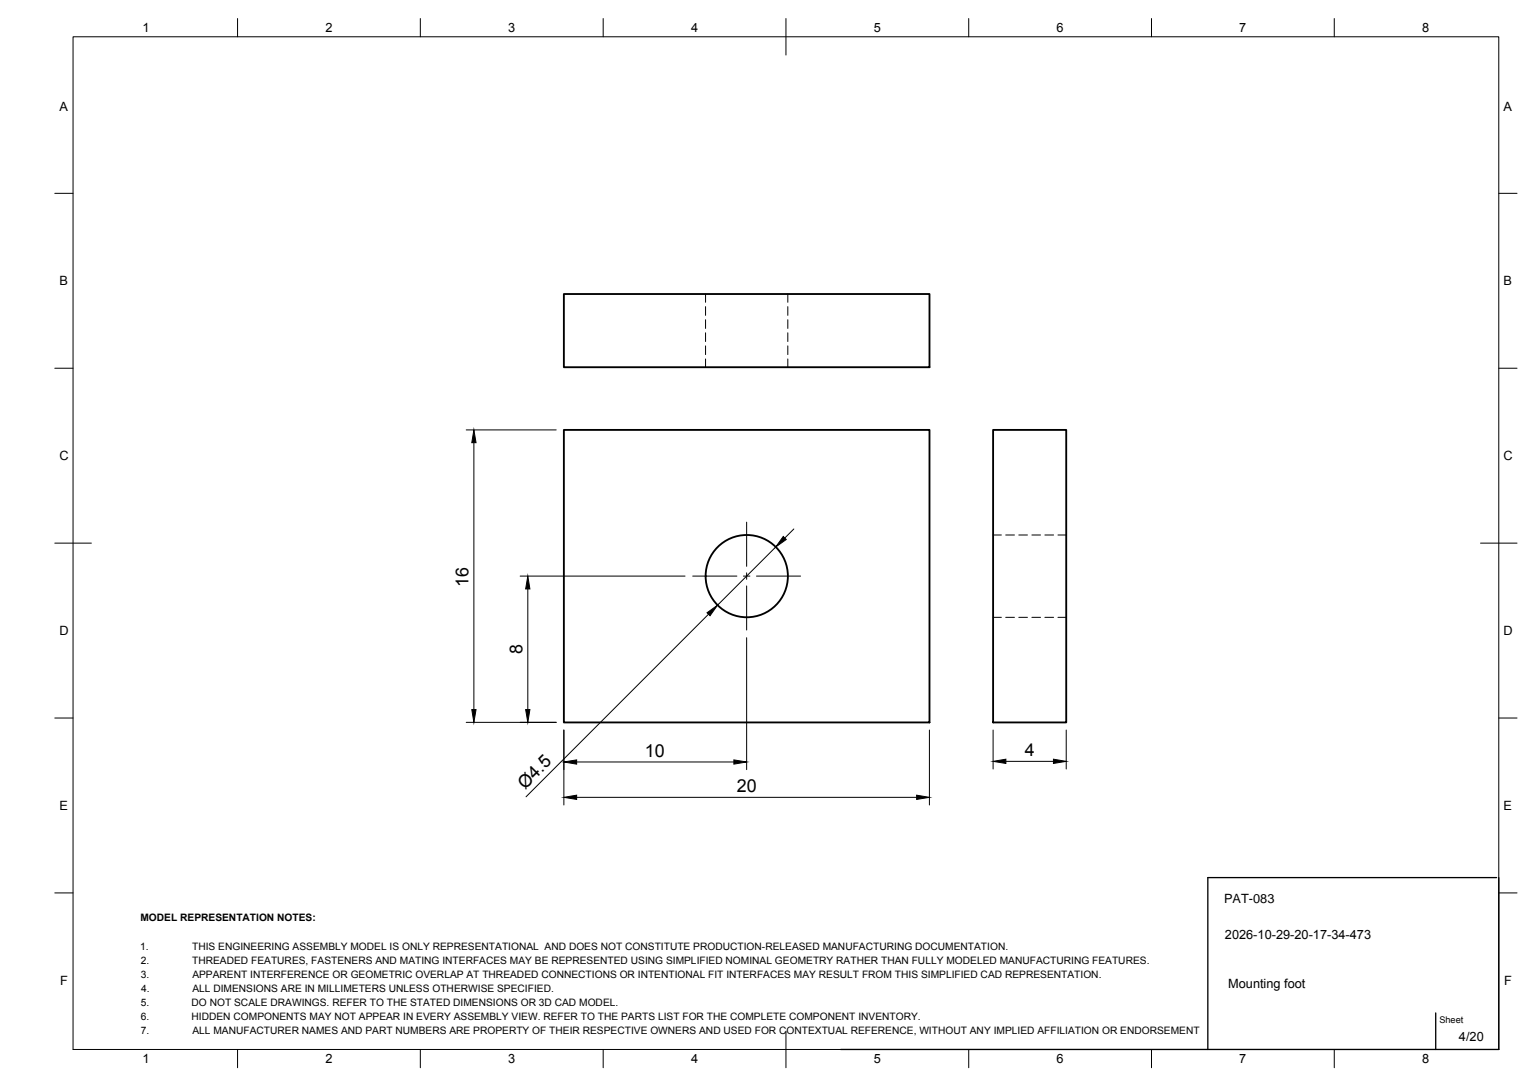
ISO-10303-21;
HEADER;
/* Generated by software containing ST-Developer
 * from STEP Tools, Inc. (www.steptools.com) 
 */

FILE_DESCRIPTION(
/* description */ ('PAT-083'),
/* implementation_level */ '2;1');

FILE_NAME(
/* name */ 'Mounting foot.step',
/* time_stamp */ '2026-10-29T20:18:00-07:00',
/* author */ (''),
/* organization */ (''),
/* preprocessor_version */ 'ST-DEVELOPER v20.2',
/* originating_system */ 'Autodesk Translation Framework v15.17.0.0',
/* authorisation */ '');

FILE_SCHEMA (('AUTOMOTIVE_DESIGN { 1 0 10303 214 3 1 1 }'));
ENDSEC;

DATA;
#10=MECHANICAL_DESIGN_GEOMETRIC_PRESENTATION_REPRESENTATION('',(#230),#8428);
#182=SHAPE_REPRESENTATION_RELATIONSHIP('SRR','None',#8516,#206);
#206=ADVANCED_BREP_SHAPE_REPRESENTATION('',(#254),#8405);
#230=STYLED_ITEM('',(#8698),#254);
#254=MANIFOLD_SOLID_BREP('Body1',#3676);
#279=FACE_BOUND('',#746,.T.);
#280=FACE_BOUND('',#748,.T.);
#362=PLANE('',#3984);
#363=PLANE('',#3985);
#364=PLANE('',#3986);
#365=PLANE('',#3987);
#366=PLANE('',#3988);
#367=PLANE('',#3989);
#503=FACE_OUTER_BOUND('',#740,.T.);
#504=FACE_OUTER_BOUND('',#741,.T.);
#505=FACE_OUTER_BOUND('',#742,.T.);
#506=FACE_OUTER_BOUND('',#743,.T.);
#507=FACE_OUTER_BOUND('',#744,.T.);
#508=FACE_OUTER_BOUND('',#745,.T.);
#509=FACE_OUTER_BOUND('',#747,.T.);
#740=EDGE_LOOP('',(#2494,#2495,#2496,#2497));
#741=EDGE_LOOP('',(#2498,#2499,#2500,#2501));
#742=EDGE_LOOP('',(#2502,#2503,#2504,#2505));
#743=EDGE_LOOP('',(#2506,#2507,#2508,#2509));
#744=EDGE_LOOP('',(#2510,#2511,#2512,#2513));
#745=EDGE_LOOP('',(#2514,#2515,#2516,#2517));
#746=EDGE_LOOP('',(#2518));
#747=EDGE_LOOP('',(#2519,#2520,#2521,#2522));
#748=EDGE_LOOP('',(#2523));
#1056=LINE('',#5665,#1300);
#1057=LINE('',#5670,#1301);
#1058=LINE('',#5672,#1302);
#1059=LINE('',#5674,#1303);
#1060=LINE('',#5675,#1304);
#1061=LINE('',#5678,#1305);
#1062=LINE('',#5680,#1306);
#1063=LINE('',#5681,#1307);
#1064=LINE('',#5684,#1308);
#1065=LINE('',#5686,#1309);
#1066=LINE('',#5687,#1310);
#1067=LINE('',#5689,#1311);
#1068=LINE('',#5690,#1312);
#1300=VECTOR('',#4484,0.225);
#1301=VECTOR('',#4489,1.);
#1302=VECTOR('',#4490,1.);
#1303=VECTOR('',#4491,1.);
#1304=VECTOR('',#4492,1.);
#1305=VECTOR('',#4495,1.);
#1306=VECTOR('',#4496,1.);
#1307=VECTOR('',#4497,1.);
#1308=VECTOR('',#4500,1.);
#1309=VECTOR('',#4501,1.);
#1310=VECTOR('',#4502,1.);
#1311=VECTOR('',#4505,1.);
#1312=VECTOR('',#4506,1.);
#1534=CIRCLE('',#3982,0.225);
#1535=CIRCLE('',#3983,0.225);
#1725=VERTEX_POINT('',#5662);
#1726=VERTEX_POINT('',#5664);
#1727=VERTEX_POINT('',#5668);
#1728=VERTEX_POINT('',#5669);
#1729=VERTEX_POINT('',#5671);
#1730=VERTEX_POINT('',#5673);
#1731=VERTEX_POINT('',#5677);
#1732=VERTEX_POINT('',#5679);
#1733=VERTEX_POINT('',#5683);
#1734=VERTEX_POINT('',#5685);
#2023=EDGE_CURVE('',#1725,#1725,#1534,.T.);
#2024=EDGE_CURVE('',#1725,#1726,#1056,.T.);
#2025=EDGE_CURVE('',#1726,#1726,#1535,.T.);
#2026=EDGE_CURVE('',#1727,#1728,#1057,.T.);
#2027=EDGE_CURVE('',#1728,#1729,#1058,.T.);
#2028=EDGE_CURVE('',#1730,#1729,#1059,.T.);
#2029=EDGE_CURVE('',#1727,#1730,#1060,.T.);
#2030=EDGE_CURVE('',#1731,#1727,#1061,.T.);
#2031=EDGE_CURVE('',#1732,#1730,#1062,.T.);
#2032=EDGE_CURVE('',#1731,#1732,#1063,.T.);
#2033=EDGE_CURVE('',#1733,#1731,#1064,.T.);
#2034=EDGE_CURVE('',#1734,#1732,#1065,.T.);
#2035=EDGE_CURVE('',#1733,#1734,#1066,.T.);
#2036=EDGE_CURVE('',#1728,#1733,#1067,.T.);
#2037=EDGE_CURVE('',#1729,#1734,#1068,.T.);
#2494=ORIENTED_EDGE('',*,*,#2023,.F.);
#2495=ORIENTED_EDGE('',*,*,#2024,.T.);
#2496=ORIENTED_EDGE('',*,*,#2025,.F.);
#2497=ORIENTED_EDGE('',*,*,#2024,.F.);
#2498=ORIENTED_EDGE('',*,*,#2026,.T.);
#2499=ORIENTED_EDGE('',*,*,#2027,.T.);
#2500=ORIENTED_EDGE('',*,*,#2028,.F.);
#2501=ORIENTED_EDGE('',*,*,#2029,.F.);
#2502=ORIENTED_EDGE('',*,*,#2030,.T.);
#2503=ORIENTED_EDGE('',*,*,#2029,.T.);
#2504=ORIENTED_EDGE('',*,*,#2031,.F.);
#2505=ORIENTED_EDGE('',*,*,#2032,.F.);
#2506=ORIENTED_EDGE('',*,*,#2033,.T.);
#2507=ORIENTED_EDGE('',*,*,#2032,.T.);
#2508=ORIENTED_EDGE('',*,*,#2034,.F.);
#2509=ORIENTED_EDGE('',*,*,#2035,.F.);
#2510=ORIENTED_EDGE('',*,*,#2036,.T.);
#2511=ORIENTED_EDGE('',*,*,#2035,.T.);
#2512=ORIENTED_EDGE('',*,*,#2037,.F.);
#2513=ORIENTED_EDGE('',*,*,#2027,.F.);
#2514=ORIENTED_EDGE('',*,*,#2037,.T.);
#2515=ORIENTED_EDGE('',*,*,#2034,.T.);
#2516=ORIENTED_EDGE('',*,*,#2031,.T.);
#2517=ORIENTED_EDGE('',*,*,#2028,.T.);
#2518=ORIENTED_EDGE('',*,*,#2025,.T.);
#2519=ORIENTED_EDGE('',*,*,#2036,.F.);
#2520=ORIENTED_EDGE('',*,*,#2026,.F.);
#2521=ORIENTED_EDGE('',*,*,#2030,.F.);
#2522=ORIENTED_EDGE('',*,*,#2033,.F.);
#2523=ORIENTED_EDGE('',*,*,#2023,.T.);
#3366=CYLINDRICAL_SURFACE('',#3981,0.225);
#3450=ADVANCED_FACE('',(#503),#3366,.F.);
#3451=ADVANCED_FACE('',(#504),#362,.T.);
#3452=ADVANCED_FACE('',(#505),#363,.T.);
#3453=ADVANCED_FACE('',(#506),#364,.T.);
#3454=ADVANCED_FACE('',(#507),#365,.T.);
#3455=ADVANCED_FACE('',(#508,#279),#366,.T.);
#3456=ADVANCED_FACE('',(#509,#280),#367,.F.);
#3676=CLOSED_SHELL('',(#3450,#3451,#3452,#3453,#3454,#3455,#3456));
#3980=AXIS2_PLACEMENT_3D('',#5660,#4478,#4479);
#3981=AXIS2_PLACEMENT_3D('',#5661,#4480,#4481);
#3982=AXIS2_PLACEMENT_3D('',#5663,#4482,#4483);
#3983=AXIS2_PLACEMENT_3D('',#5666,#4485,#4486);
#3984=AXIS2_PLACEMENT_3D('',#5667,#4487,#4488);
#3985=AXIS2_PLACEMENT_3D('',#5676,#4493,#4494);
#3986=AXIS2_PLACEMENT_3D('',#5682,#4498,#4499);
#3987=AXIS2_PLACEMENT_3D('',#5688,#4503,#4504);
#3988=AXIS2_PLACEMENT_3D('',#5691,#4507,#4508);
#3989=AXIS2_PLACEMENT_3D('',#5692,#4509,#4510);
#4478=DIRECTION('axis',(0.,0.,1.));
#4479=DIRECTION('refdir',(1.,0.,0.));
#4480=DIRECTION('center_axis',(0.,0.,1.));
#4481=DIRECTION('ref_axis',(1.,0.,0.));
#4482=DIRECTION('center_axis',(0.,0.,1.));
#4483=DIRECTION('ref_axis',(1.,0.,0.));
#4484=DIRECTION('',(0.,0.,1.));
#4485=DIRECTION('center_axis',(0.,0.,-1.));
#4486=DIRECTION('ref_axis',(1.,0.,0.));
#4487=DIRECTION('center_axis',(0.,1.,0.));
#4488=DIRECTION('ref_axis',(-1.,0.,0.));
#4489=DIRECTION('',(-1.,0.,0.));
#4490=DIRECTION('',(0.,0.,1.));
#4491=DIRECTION('',(-1.,0.,0.));
#4492=DIRECTION('',(0.,0.,1.));
#4493=DIRECTION('center_axis',(1.,0.,0.));
#4494=DIRECTION('ref_axis',(0.,1.,0.));
#4495=DIRECTION('',(0.,1.,0.));
#4496=DIRECTION('',(0.,1.,0.));
#4497=DIRECTION('',(0.,0.,1.));
#4498=DIRECTION('center_axis',(0.,-1.,0.));
#4499=DIRECTION('ref_axis',(1.,0.,0.));
#4500=DIRECTION('',(1.,0.,0.));
#4501=DIRECTION('',(1.,0.,0.));
#4502=DIRECTION('',(0.,0.,1.));
#4503=DIRECTION('center_axis',(-1.,0.,0.));
#4504=DIRECTION('ref_axis',(0.,-1.,0.));
#4505=DIRECTION('',(0.,-1.,0.));
#4506=DIRECTION('',(0.,-1.,0.));
#4507=DIRECTION('center_axis',(0.,0.,1.));
#4508=DIRECTION('ref_axis',(1.,0.,0.));
#4509=DIRECTION('center_axis',(0.,0.,1.));
#4510=DIRECTION('ref_axis',(1.,0.,0.));
#5660=CARTESIAN_POINT('',(0.,0.,0.));
#5661=CARTESIAN_POINT('Origin',(0.,-3.,0.5));
#5662=CARTESIAN_POINT('',(-0.225,-3.,0.6));
#5663=CARTESIAN_POINT('Origin',(0.,-3.,0.6));
#5664=CARTESIAN_POINT('',(-0.225,-3.,1.));
#5665=CARTESIAN_POINT('',(-0.225,-3.,0.5));
#5666=CARTESIAN_POINT('Origin',(0.,-3.,1.));
#5667=CARTESIAN_POINT('Origin',(1.,-2.2,0.6));
#5668=CARTESIAN_POINT('',(1.,-2.2,0.6));
#5669=CARTESIAN_POINT('',(-1.,-2.2,0.6));
#5670=CARTESIAN_POINT('',(1.,-2.2,0.6));
#5671=CARTESIAN_POINT('',(-1.,-2.2,1.));
#5672=CARTESIAN_POINT('',(-1.,-2.2,0.6));
#5673=CARTESIAN_POINT('',(1.,-2.2,1.));
#5674=CARTESIAN_POINT('',(1.,-2.2,1.));
#5675=CARTESIAN_POINT('',(1.,-2.2,0.6));
#5676=CARTESIAN_POINT('Origin',(1.,-3.8,0.6));
#5677=CARTESIAN_POINT('',(1.,-3.8,0.6));
#5678=CARTESIAN_POINT('',(1.,-3.8,0.6));
#5679=CARTESIAN_POINT('',(1.,-3.8,1.));
#5680=CARTESIAN_POINT('',(1.,-3.8,1.));
#5681=CARTESIAN_POINT('',(1.,-3.8,0.6));
#5682=CARTESIAN_POINT('Origin',(-1.,-3.8,0.6));
#5683=CARTESIAN_POINT('',(-1.,-3.8,0.6));
#5684=CARTESIAN_POINT('',(-1.,-3.8,0.6));
#5685=CARTESIAN_POINT('',(-1.,-3.8,1.));
#5686=CARTESIAN_POINT('',(-1.,-3.8,1.));
#5687=CARTESIAN_POINT('',(-1.,-3.8,0.6));
#5688=CARTESIAN_POINT('Origin',(-1.,-2.2,0.6));
#5689=CARTESIAN_POINT('',(-1.,-2.2,0.6));
#5690=CARTESIAN_POINT('',(-1.,-2.2,1.));
#5691=CARTESIAN_POINT('Origin',(0.,-3.,1.));
#5692=CARTESIAN_POINT('Origin',(0.,-3.,0.6));
#8379=UNCERTAINTY_MEASURE_WITH_UNIT(LENGTH_MEASURE(0.001),#8429,
'DISTANCE_ACCURACY_VALUE',
'Maximum model space distance between geometric entities at asserted c
onnectivities');
#8402=UNCERTAINTY_MEASURE_WITH_UNIT(LENGTH_MEASURE(0.001),#8429,
'DISTANCE_ACCURACY_VALUE',
'Maximum model space distance between geometric entities at asserted c
onnectivities');
#8405=(
GEOMETRIC_REPRESENTATION_CONTEXT(3)
GLOBAL_UNCERTAINTY_ASSIGNED_CONTEXT((#8379))
GLOBAL_UNIT_ASSIGNED_CONTEXT((#8429,#8431,#8432))
REPRESENTATION_CONTEXT('','3D')
);
#8428=(
GEOMETRIC_REPRESENTATION_CONTEXT(3)
GLOBAL_UNCERTAINTY_ASSIGNED_CONTEXT((#8402))
GLOBAL_UNIT_ASSIGNED_CONTEXT((#8429,#8431,#8432))
REPRESENTATION_CONTEXT('','3D')
);
#8429=(
LENGTH_UNIT()
NAMED_UNIT(*)
SI_UNIT(.CENTI.,.METRE.)
);
#8431=(
NAMED_UNIT(*)
PLANE_ANGLE_UNIT()
SI_UNIT($,.RADIAN.)
);
#8432=(
NAMED_UNIT(*)
SI_UNIT($,.STERADIAN.)
SOLID_ANGLE_UNIT()
);
#8435=SHAPE_DEFINITION_REPRESENTATION(#8460,#8516);
#8460=PRODUCT_DEFINITION_SHAPE('',$,#8542);
#8516=SHAPE_REPRESENTATION('',(#3980),#8405);
#8539=PRODUCT_DEFINITION_CONTEXT('part definition',#8616,'design');
#8542=PRODUCT_DEFINITION('Mounting foot','Mounting foot',#8567,
#8539);
#8567=PRODUCT_DEFINITION_FORMATION('',$,#8620);
#8616=APPLICATION_CONTEXT(
'Core Data for Automotive Mechanical Design Process');
#8617=PRODUCT_CONTEXT('part definition',#8616,'mechanical');
#8620=PRODUCT('Mounting foot','Mounting foot',
'Mounting foot',(#8617));
#8692=COLOUR_RGB('Sky Blue',0.24,0.69,0.87);
#8693=FILL_AREA_STYLE_COLOUR('',#8692);
#8694=FILL_AREA_STYLE('',(#8693));
#8695=SURFACE_STYLE_FILL_AREA(#8694);
#8696=SURFACE_SIDE_STYLE('',(#8695));
#8697=SURFACE_STYLE_USAGE(.BOTH.,#8696);
#8698=PRESENTATION_STYLE_ASSIGNMENT((#8697));
ENDSEC;
END-ISO-10303-21;
